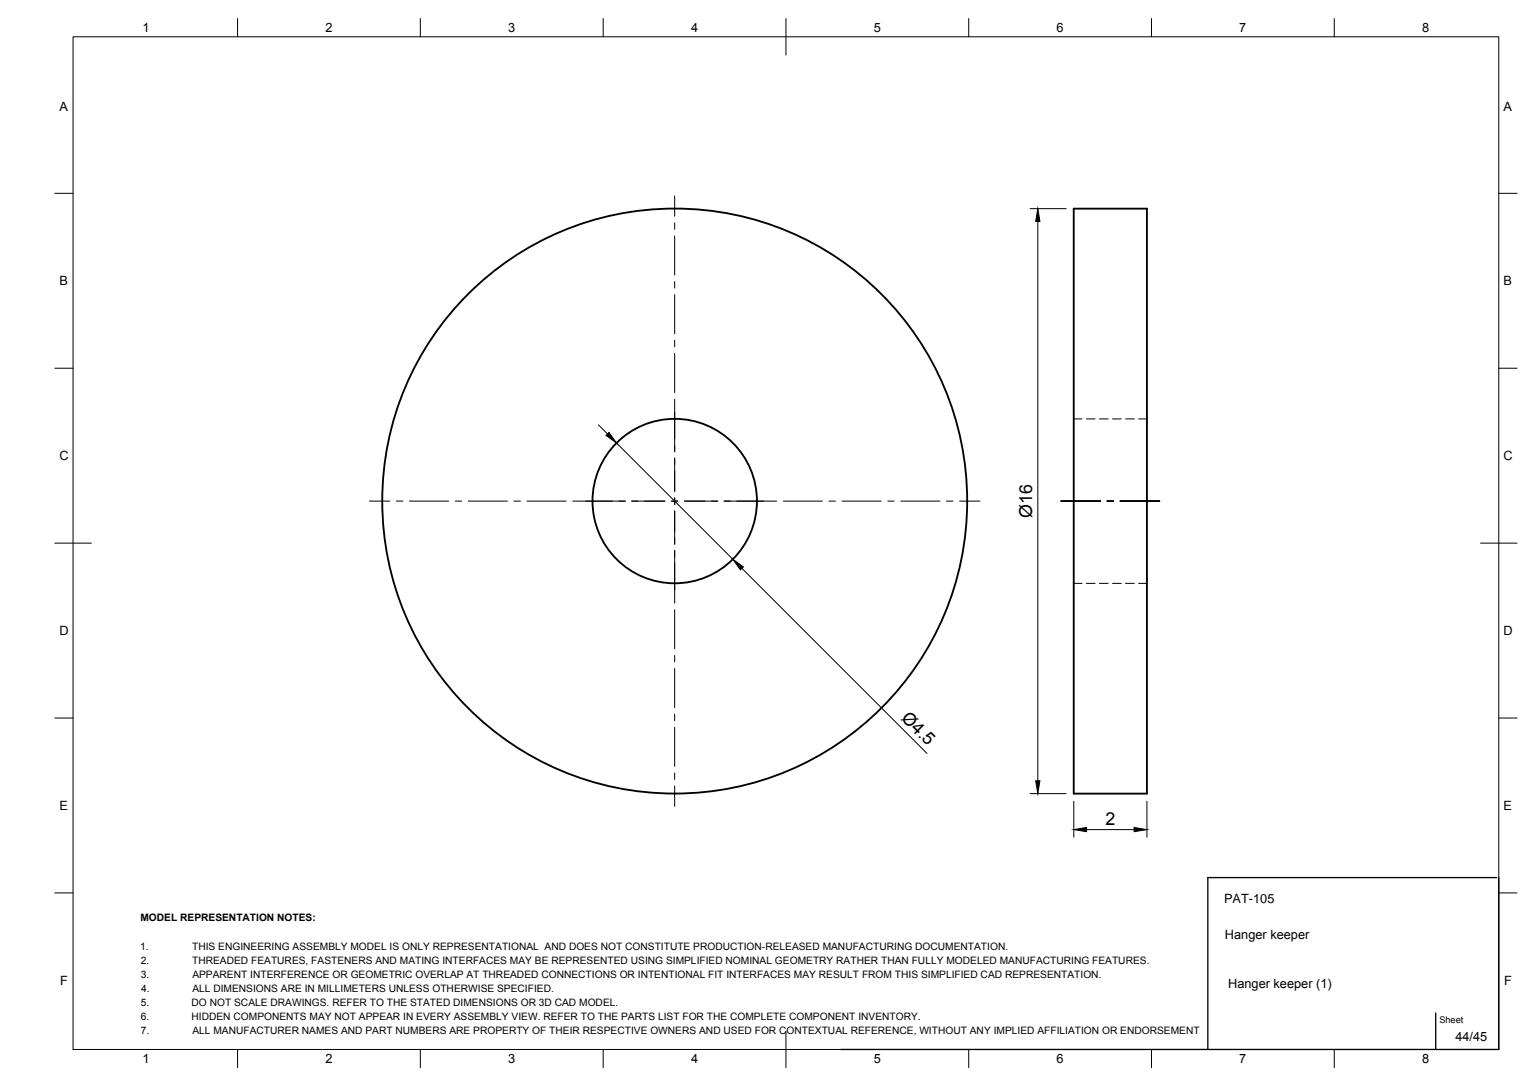
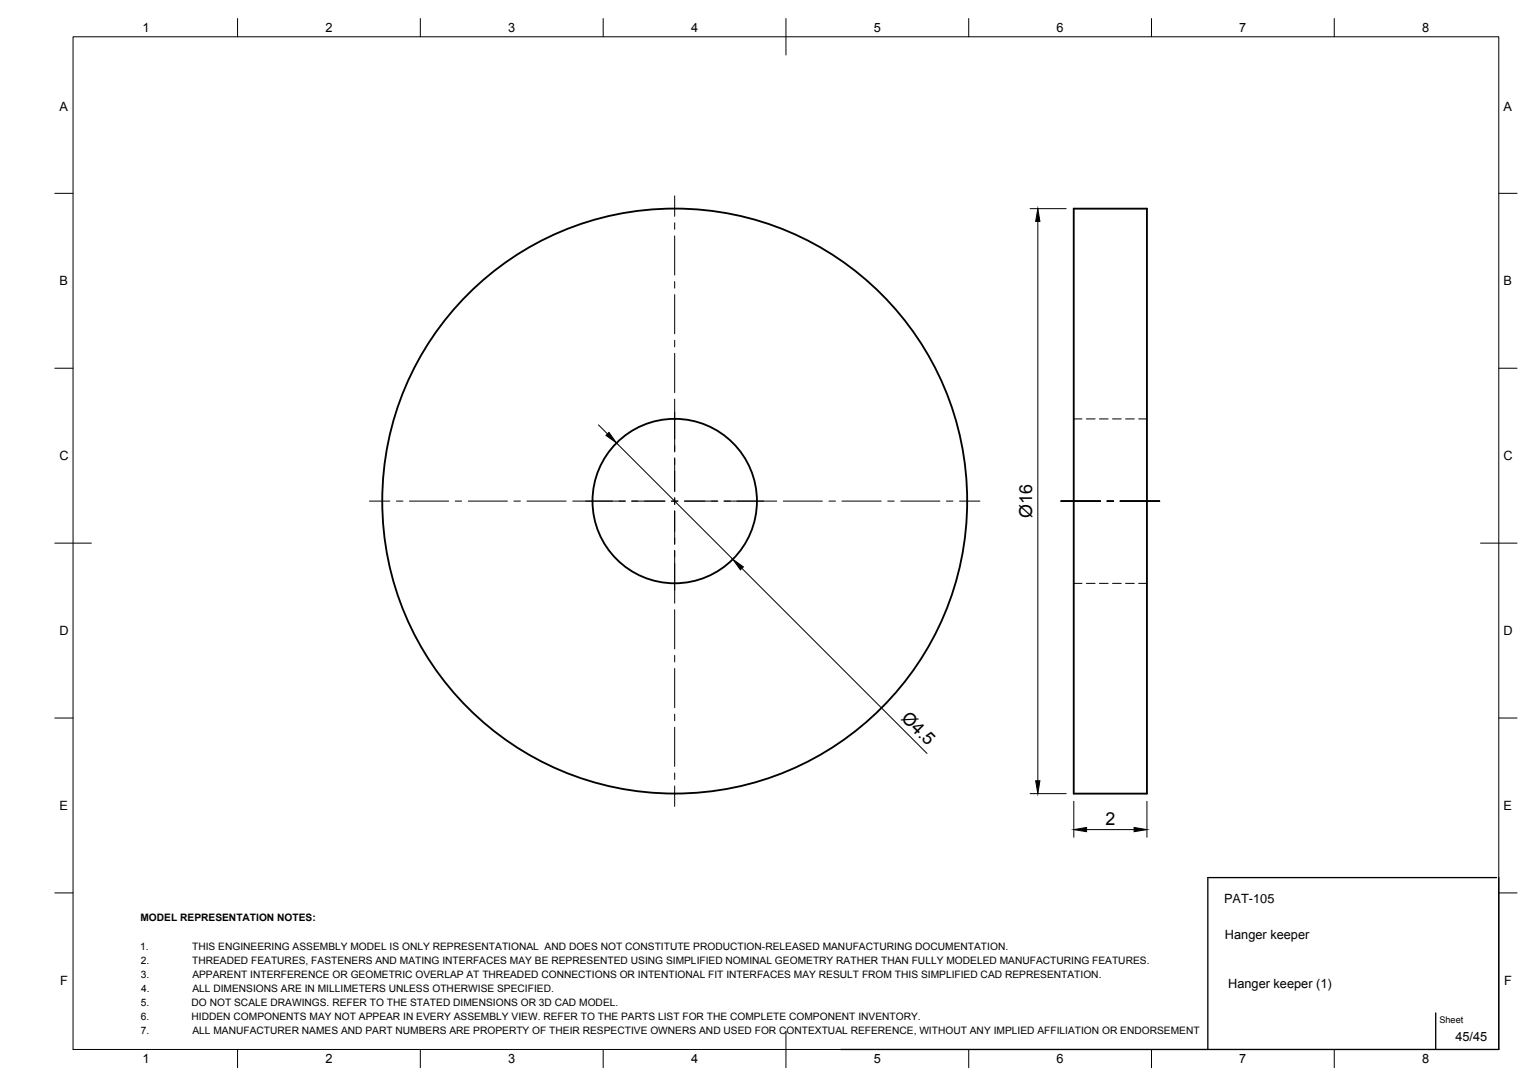
ISO-10303-21;
HEADER;
/* Generated by software containing ST-Developer
 * from STEP Tools, Inc. (www.steptools.com) 
 */

FILE_DESCRIPTION(
/* description */ ('Torque wrench calibration arm'),
/* implementation_level */ '2;1');

FILE_NAME(
/* name */ 'Hanger keeper.step',
/* time_stamp */ '2026-10-28T03:24:52-07:00',
/* author */ (''),
/* organization */ (''),
/* preprocessor_version */ 'ST-DEVELOPER v20.2',
/* originating_system */ 'Autodesk Translation Framework v15.17.0.0',
/* authorisation */ '');

FILE_SCHEMA (('AUTOMOTIVE_DESIGN { 1 0 10303 214 3 1 1 }'));
ENDSEC;

DATA;
#10=MECHANICAL_DESIGN_GEOMETRIC_PRESENTATION_REPRESENTATION('',(#477),#12783);
#386=SHAPE_REPRESENTATION_RELATIONSHIP('SRR','None',#12971,#423);
#423=ADVANCED_BREP_SHAPE_REPRESENTATION('',(#529),#12780);
#477=STYLED_ITEM('',(#13205),#529);
#529=MANIFOLD_SOLID_BREP('Body1',#6548);
#647=FACE_BOUND('',#1760,.T.);
#648=FACE_BOUND('',#1762,.T.);
#860=PLANE('',#7762);
#861=PLANE('',#7763);
#1246=FACE_OUTER_BOUND('',#1757,.T.);
#1247=FACE_OUTER_BOUND('',#1758,.T.);
#1248=FACE_OUTER_BOUND('',#1759,.T.);
#1249=FACE_OUTER_BOUND('',#1761,.T.);
#1757=EDGE_LOOP('',(#5903,#5904,#5905,#5906));
#1758=EDGE_LOOP('',(#5907,#5908,#5909,#5910));
#1759=EDGE_LOOP('',(#5911));
#1760=EDGE_LOOP('',(#5912));
#1761=EDGE_LOOP('',(#5913));
#1762=EDGE_LOOP('',(#5914));
#2174=LINE('',#12592,#2589);
#2175=LINE('',#12598,#2590);
#2589=VECTOR('',#9794,0.225000000000001);
#2590=VECTOR('',#9801,0.799999999999997);
#2956=CIRCLE('',#7757,0.225000000000001);
#2957=CIRCLE('',#7758,0.225000000000001);
#2958=CIRCLE('',#7760,0.799999999999997);
#2959=CIRCLE('',#7761,0.799999999999997);
#3506=VERTEX_POINT('',#12589);
#3507=VERTEX_POINT('',#12591);
#3508=VERTEX_POINT('',#12595);
#3509=VERTEX_POINT('',#12597);
#4309=EDGE_CURVE('',#3506,#3506,#2956,.T.);
#4310=EDGE_CURVE('',#3506,#3507,#2174,.T.);
#4311=EDGE_CURVE('',#3507,#3507,#2957,.T.);
#4312=EDGE_CURVE('',#3508,#3508,#2958,.T.);
#4313=EDGE_CURVE('',#3508,#3509,#2175,.T.);
#4314=EDGE_CURVE('',#3509,#3509,#2959,.T.);
#5903=ORIENTED_EDGE('',*,*,#4309,.F.);
#5904=ORIENTED_EDGE('',*,*,#4310,.T.);
#5905=ORIENTED_EDGE('',*,*,#4311,.T.);
#5906=ORIENTED_EDGE('',*,*,#4310,.F.);
#5907=ORIENTED_EDGE('',*,*,#4312,.F.);
#5908=ORIENTED_EDGE('',*,*,#4313,.T.);
#5909=ORIENTED_EDGE('',*,*,#4314,.T.);
#5910=ORIENTED_EDGE('',*,*,#4313,.F.);
#5911=ORIENTED_EDGE('',*,*,#4312,.T.);
#5912=ORIENTED_EDGE('',*,*,#4309,.T.);
#5913=ORIENTED_EDGE('',*,*,#4314,.F.);
#5914=ORIENTED_EDGE('',*,*,#4311,.F.);
#6094=CYLINDRICAL_SURFACE('',#7756,0.225000000000001);
#6095=CYLINDRICAL_SURFACE('',#7759,0.799999999999997);
#6471=ADVANCED_FACE('',(#1246),#6094,.F.);
#6472=ADVANCED_FACE('',(#1247),#6095,.T.);
#6473=ADVANCED_FACE('',(#1248,#647),#860,.T.);
#6474=ADVANCED_FACE('',(#1249,#648),#861,.F.);
#6548=CLOSED_SHELL('',(#6471,#6472,#6473,#6474));
#7755=AXIS2_PLACEMENT_3D('',#12587,#9788,#9789);
#7756=AXIS2_PLACEMENT_3D('',#12588,#9790,#9791);
#7757=AXIS2_PLACEMENT_3D('',#12590,#9792,#9793);
#7758=AXIS2_PLACEMENT_3D('',#12593,#9795,#9796);
#7759=AXIS2_PLACEMENT_3D('',#12594,#9797,#9798);
#7760=AXIS2_PLACEMENT_3D('',#12596,#9799,#9800);
#7761=AXIS2_PLACEMENT_3D('',#12599,#9802,#9803);
#7762=AXIS2_PLACEMENT_3D('',#12600,#9804,#9805);
#7763=AXIS2_PLACEMENT_3D('',#12601,#9806,#9807);
#9788=DIRECTION('axis',(0.,0.,1.));
#9789=DIRECTION('refdir',(1.,0.,0.));
#9790=DIRECTION('center_axis',(0.,1.,0.));
#9791=DIRECTION('ref_axis',(1.,0.,0.));
#9792=DIRECTION('center_axis',(0.,-1.,0.));
#9793=DIRECTION('ref_axis',(1.,0.,0.));
#9794=DIRECTION('',(0.,-1.,0.));
#9795=DIRECTION('center_axis',(0.,-1.,0.));
#9796=DIRECTION('ref_axis',(1.,0.,0.));
#9797=DIRECTION('center_axis',(0.,1.,0.));
#9798=DIRECTION('ref_axis',(1.,0.,0.));
#9799=DIRECTION('center_axis',(0.,1.,0.));
#9800=DIRECTION('ref_axis',(1.,0.,0.));
#9801=DIRECTION('',(0.,-1.,0.));
#9802=DIRECTION('center_axis',(0.,1.,0.));
#9803=DIRECTION('ref_axis',(1.,0.,0.));
#9804=DIRECTION('center_axis',(0.,1.,0.));
#9805=DIRECTION('ref_axis',(1.,0.,0.));
#9806=DIRECTION('center_axis',(0.,1.,0.));
#9807=DIRECTION('ref_axis',(1.,0.,0.));
#12587=CARTESIAN_POINT('',(0.,0.,0.));
#12588=CARTESIAN_POINT('Origin',(50.,6.4,8.));
#12589=CARTESIAN_POINT('',(49.775,6.6,8.));
#12590=CARTESIAN_POINT('Origin',(50.,6.6,8.));
#12591=CARTESIAN_POINT('',(49.775,6.4,8.));
#12592=CARTESIAN_POINT('',(49.775,6.4,8.));
#12593=CARTESIAN_POINT('Origin',(50.,6.4,8.));
#12594=CARTESIAN_POINT('Origin',(50.,6.4,8.));
#12595=CARTESIAN_POINT('',(49.2,6.6,8.));
#12596=CARTESIAN_POINT('Origin',(50.,6.6,8.));
#12597=CARTESIAN_POINT('',(49.2,6.4,8.));
#12598=CARTESIAN_POINT('',(49.2,6.4,8.));
#12599=CARTESIAN_POINT('Origin',(50.,6.4,8.));
#12600=CARTESIAN_POINT('Origin',(50.,6.6,8.));
#12601=CARTESIAN_POINT('Origin',(50.,6.4,8.));
#12736=UNCERTAINTY_MEASURE_WITH_UNIT(LENGTH_MEASURE(0.001),#12784,
'DISTANCE_ACCURACY_VALUE',
'Maximum model space distance between geometric entities at asserted c
onnectivities');
#12739=UNCERTAINTY_MEASURE_WITH_UNIT(LENGTH_MEASURE(0.001),#12784,
'DISTANCE_ACCURACY_VALUE',
'Maximum model space distance between geometric entities at asserted c
onnectivities');
#12780=(
GEOMETRIC_REPRESENTATION_CONTEXT(3)
GLOBAL_UNCERTAINTY_ASSIGNED_CONTEXT((#12736))
GLOBAL_UNIT_ASSIGNED_CONTEXT((#12784,#12786,#12787))
REPRESENTATION_CONTEXT('','3D')
);
#12783=(
GEOMETRIC_REPRESENTATION_CONTEXT(3)
GLOBAL_UNCERTAINTY_ASSIGNED_CONTEXT((#12739))
GLOBAL_UNIT_ASSIGNED_CONTEXT((#12784,#12786,#12787))
REPRESENTATION_CONTEXT('','3D')
);
#12784=(
LENGTH_UNIT()
NAMED_UNIT(*)
SI_UNIT(.CENTI.,.METRE.)
);
#12786=(
NAMED_UNIT(*)
PLANE_ANGLE_UNIT()
SI_UNIT($,.RADIAN.)
);
#12787=(
NAMED_UNIT(*)
SI_UNIT($,.STERADIAN.)
SOLID_ANGLE_UNIT()
);
#12828=SHAPE_DEFINITION_REPRESENTATION(#12915,#12971);
#12915=PRODUCT_DEFINITION_SHAPE('',$,#13015);
#12971=SHAPE_REPRESENTATION('',(#7755),#12780);
#12974=PRODUCT_DEFINITION_CONTEXT('part definition',#13105,'design');
#13015=PRODUCT_DEFINITION('Hanger keeper','Hanger keeper',#13058,#12974);
#13058=PRODUCT_DEFINITION_FORMATION('',$,#13147);
#13105=APPLICATION_CONTEXT(
'Core Data for Automotive Mechanical Design Process');
#13106=PRODUCT_CONTEXT('part definition',#13105,'mechanical');
#13147=PRODUCT('Hanger keeper','Hanger keeper','Hanger keeper',(#13106));
#13199=COLOUR_RGB('Sky Blue',0.24,0.69,0.87);
#13200=FILL_AREA_STYLE_COLOUR('',#13199);
#13201=FILL_AREA_STYLE('',(#13200));
#13202=SURFACE_STYLE_FILL_AREA(#13201);
#13203=SURFACE_SIDE_STYLE('',(#13202));
#13204=SURFACE_STYLE_USAGE(.BOTH.,#13203);
#13205=PRESENTATION_STYLE_ASSIGNMENT((#13204));
ENDSEC;
END-ISO-10303-21;
